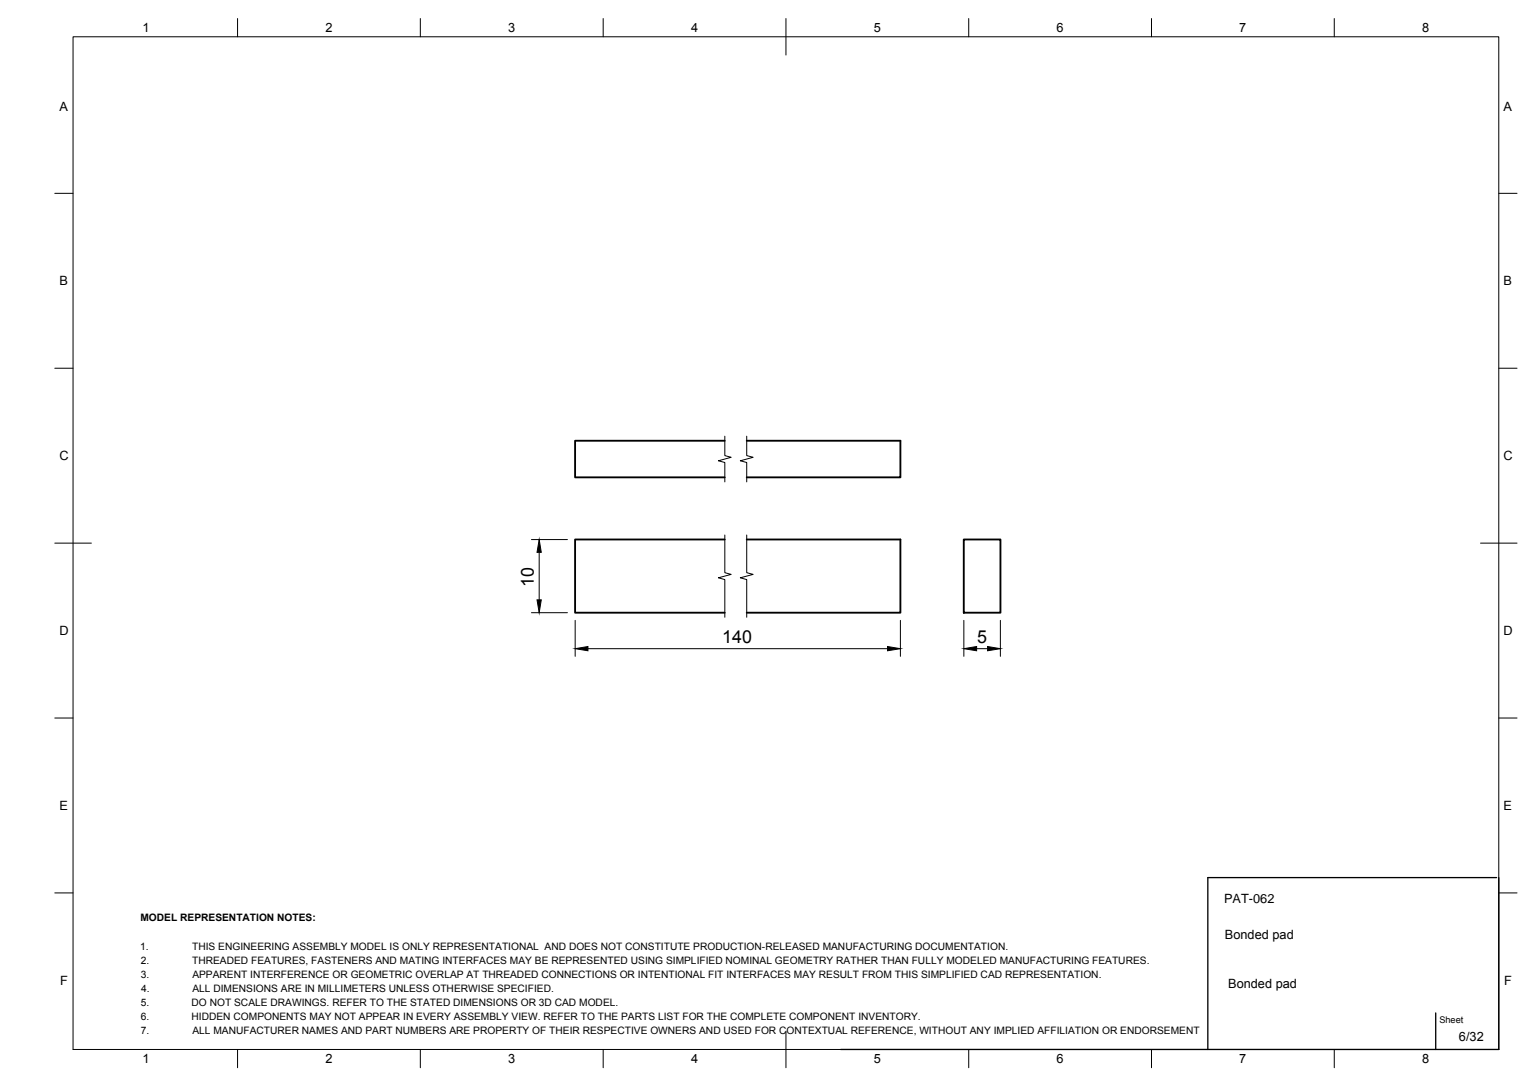
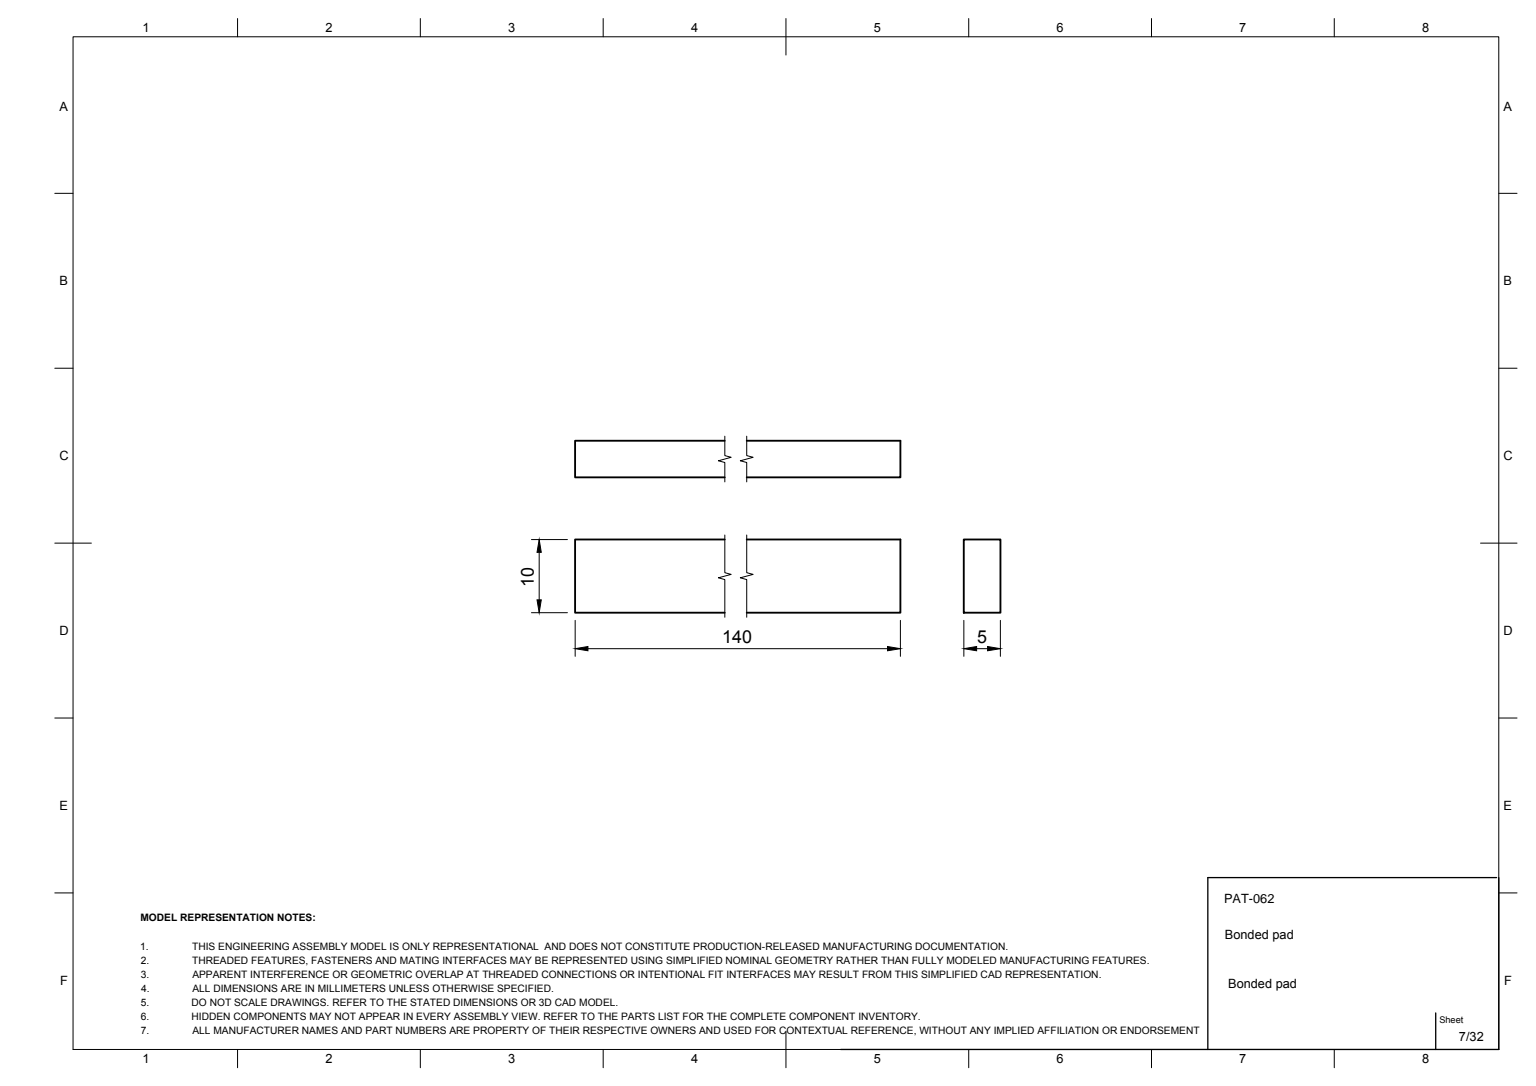
ISO-10303-21;
HEADER;
/* Generated by software containing ST-Developer
 * from STEP Tools, Inc. (www.steptools.com) 
 */

FILE_DESCRIPTION(
/* description */ ('Jaw-coupled motor to shaft test stand'),
/* implementation_level */ '2;1');

FILE_NAME(
/* name */ 'Bonded pad.step',
/* time_stamp */ '2026-10-27T10:46:06-07:00',
/* author */ (''),
/* organization */ (''),
/* preprocessor_version */ 'ST-DEVELOPER v20.2',
/* originating_system */ 'Autodesk Translation Framework v15.17.0.0',
/* authorisation */ '');

FILE_SCHEMA (('AUTOMOTIVE_DESIGN { 1 0 10303 214 3 1 1 }'));
ENDSEC;

DATA;
#10=MECHANICAL_DESIGN_GEOMETRIC_PRESENTATION_REPRESENTATION('',(#341),#19361);
#277=SHAPE_REPRESENTATION_RELATIONSHIP('SRR','None',#19491,#309);
#309=ADVANCED_BREP_SHAPE_REPRESENTATION('',(#374),#19327);
#341=STYLED_ITEM('',(#19760),#374);
#374=MANIFOLD_SOLID_BREP('Body1',#10985);
#522=PLANE('',#11401);
#523=PLANE('',#11402);
#524=PLANE('',#11403);
#525=PLANE('',#11404);
#526=PLANE('',#11405);
#527=PLANE('',#11406);
#1034=FACE_OUTER_BOUND('',#1666,.T.);
#1035=FACE_OUTER_BOUND('',#1667,.T.);
#1036=FACE_OUTER_BOUND('',#1668,.T.);
#1037=FACE_OUTER_BOUND('',#1669,.T.);
#1038=FACE_OUTER_BOUND('',#1670,.T.);
#1039=FACE_OUTER_BOUND('',#1671,.T.);
#1666=EDGE_LOOP('',(#7406,#7407,#7408,#7409));
#1667=EDGE_LOOP('',(#7410,#7411,#7412,#7413));
#1668=EDGE_LOOP('',(#7414,#7415,#7416,#7417));
#1669=EDGE_LOOP('',(#7418,#7419,#7420,#7421));
#1670=EDGE_LOOP('',(#7422,#7423,#7424,#7425));
#1671=EDGE_LOOP('',(#7426,#7427,#7428,#7429));
#2393=LINE('',#15496,#3546);
#2394=LINE('',#15498,#3547);
#2395=LINE('',#15500,#3548);
#2396=LINE('',#15501,#3549);
#2397=LINE('',#15504,#3550);
#2398=LINE('',#15506,#3551);
#2399=LINE('',#15507,#3552);
#2400=LINE('',#15510,#3553);
#2401=LINE('',#15512,#3554);
#2402=LINE('',#15513,#3555);
#2403=LINE('',#15515,#3556);
#2404=LINE('',#15516,#3557);
#3546=VECTOR('',#12416,1.);
#3547=VECTOR('',#12417,1.);
#3548=VECTOR('',#12418,1.);
#3549=VECTOR('',#12419,1.);
#3550=VECTOR('',#12422,1.);
#3551=VECTOR('',#12423,1.);
#3552=VECTOR('',#12424,1.);
#3553=VECTOR('',#12427,1.);
#3554=VECTOR('',#12428,1.);
#3555=VECTOR('',#12429,1.);
#3556=VECTOR('',#12432,1.);
#3557=VECTOR('',#12433,1.);
#4963=VERTEX_POINT('',#15494);
#4964=VERTEX_POINT('',#15495);
#4965=VERTEX_POINT('',#15497);
#4966=VERTEX_POINT('',#15499);
#4967=VERTEX_POINT('',#15503);
#4968=VERTEX_POINT('',#15505);
#4969=VERTEX_POINT('',#15509);
#4970=VERTEX_POINT('',#15511);
#5914=EDGE_CURVE('',#4963,#4964,#2393,.T.);
#5915=EDGE_CURVE('',#4964,#4965,#2394,.T.);
#5916=EDGE_CURVE('',#4966,#4965,#2395,.T.);
#5917=EDGE_CURVE('',#4963,#4966,#2396,.T.);
#5918=EDGE_CURVE('',#4967,#4963,#2397,.T.);
#5919=EDGE_CURVE('',#4968,#4966,#2398,.T.);
#5920=EDGE_CURVE('',#4967,#4968,#2399,.T.);
#5921=EDGE_CURVE('',#4969,#4967,#2400,.T.);
#5922=EDGE_CURVE('',#4970,#4968,#2401,.T.);
#5923=EDGE_CURVE('',#4969,#4970,#2402,.T.);
#5924=EDGE_CURVE('',#4964,#4969,#2403,.T.);
#5925=EDGE_CURVE('',#4965,#4970,#2404,.T.);
#7406=ORIENTED_EDGE('',*,*,#5914,.T.);
#7407=ORIENTED_EDGE('',*,*,#5915,.T.);
#7408=ORIENTED_EDGE('',*,*,#5916,.F.);
#7409=ORIENTED_EDGE('',*,*,#5917,.F.);
#7410=ORIENTED_EDGE('',*,*,#5918,.T.);
#7411=ORIENTED_EDGE('',*,*,#5917,.T.);
#7412=ORIENTED_EDGE('',*,*,#5919,.F.);
#7413=ORIENTED_EDGE('',*,*,#5920,.F.);
#7414=ORIENTED_EDGE('',*,*,#5921,.T.);
#7415=ORIENTED_EDGE('',*,*,#5920,.T.);
#7416=ORIENTED_EDGE('',*,*,#5922,.F.);
#7417=ORIENTED_EDGE('',*,*,#5923,.F.);
#7418=ORIENTED_EDGE('',*,*,#5924,.T.);
#7419=ORIENTED_EDGE('',*,*,#5923,.T.);
#7420=ORIENTED_EDGE('',*,*,#5925,.F.);
#7421=ORIENTED_EDGE('',*,*,#5915,.F.);
#7422=ORIENTED_EDGE('',*,*,#5925,.T.);
#7423=ORIENTED_EDGE('',*,*,#5922,.T.);
#7424=ORIENTED_EDGE('',*,*,#5919,.T.);
#7425=ORIENTED_EDGE('',*,*,#5916,.T.);
#7426=ORIENTED_EDGE('',*,*,#5924,.F.);
#7427=ORIENTED_EDGE('',*,*,#5914,.F.);
#7428=ORIENTED_EDGE('',*,*,#5918,.F.);
#7429=ORIENTED_EDGE('',*,*,#5921,.F.);
#10376=ADVANCED_FACE('',(#1034),#522,.T.);
#10377=ADVANCED_FACE('',(#1035),#523,.T.);
#10378=ADVANCED_FACE('',(#1036),#524,.T.);
#10379=ADVANCED_FACE('',(#1037),#525,.T.);
#10380=ADVANCED_FACE('',(#1038),#526,.T.);
#10381=ADVANCED_FACE('',(#1039),#527,.F.);
#10985=CLOSED_SHELL('',(#10376,#10377,#10378,#10379,#10380,#10381));
#11400=AXIS2_PLACEMENT_3D('',#15492,#12412,#12413);
#11401=AXIS2_PLACEMENT_3D('',#15493,#12414,#12415);
#11402=AXIS2_PLACEMENT_3D('',#15502,#12420,#12421);
#11403=AXIS2_PLACEMENT_3D('',#15508,#12425,#12426);
#11404=AXIS2_PLACEMENT_3D('',#15514,#12430,#12431);
#11405=AXIS2_PLACEMENT_3D('',#15517,#12434,#12435);
#11406=AXIS2_PLACEMENT_3D('',#15518,#12436,#12437);
#12412=DIRECTION('axis',(0.,0.,1.));
#12413=DIRECTION('refdir',(1.,0.,0.));
#12414=DIRECTION('center_axis',(0.,1.,0.));
#12415=DIRECTION('ref_axis',(-1.,0.,0.));
#12416=DIRECTION('',(-1.,0.,0.));
#12417=DIRECTION('',(0.,0.,1.));
#12418=DIRECTION('',(-1.,0.,0.));
#12419=DIRECTION('',(0.,0.,1.));
#12420=DIRECTION('center_axis',(1.,0.,0.));
#12421=DIRECTION('ref_axis',(0.,1.,0.));
#12422=DIRECTION('',(0.,1.,0.));
#12423=DIRECTION('',(0.,1.,0.));
#12424=DIRECTION('',(0.,0.,1.));
#12425=DIRECTION('center_axis',(0.,-1.,0.));
#12426=DIRECTION('ref_axis',(1.,0.,0.));
#12427=DIRECTION('',(1.,0.,0.));
#12428=DIRECTION('',(1.,0.,0.));
#12429=DIRECTION('',(0.,0.,1.));
#12430=DIRECTION('center_axis',(-1.,0.,0.));
#12431=DIRECTION('ref_axis',(0.,-1.,0.));
#12432=DIRECTION('',(0.,-1.,0.));
#12433=DIRECTION('',(0.,-1.,0.));
#12434=DIRECTION('center_axis',(0.,0.,1.));
#12435=DIRECTION('ref_axis',(1.,0.,0.));
#12436=DIRECTION('center_axis',(0.,0.,1.));
#12437=DIRECTION('ref_axis',(1.,0.,0.));
#15492=CARTESIAN_POINT('',(0.,0.,0.));
#15493=CARTESIAN_POINT('Origin',(7.,-11.5,-0.5));
#15494=CARTESIAN_POINT('',(7.,-11.5,-0.5));
#15495=CARTESIAN_POINT('',(-7.,-11.5,-0.5));
#15496=CARTESIAN_POINT('',(7.,-11.5,-0.5));
#15497=CARTESIAN_POINT('',(-7.,-11.5,0.));
#15498=CARTESIAN_POINT('',(-7.,-11.5,-0.5));
#15499=CARTESIAN_POINT('',(7.,-11.5,0.));
#15500=CARTESIAN_POINT('',(7.,-11.5,0.));
#15501=CARTESIAN_POINT('',(7.,-11.5,-0.5));
#15502=CARTESIAN_POINT('Origin',(7.,-12.5,-0.5));
#15503=CARTESIAN_POINT('',(7.,-12.5,-0.5));
#15504=CARTESIAN_POINT('',(7.,-12.5,-0.5));
#15505=CARTESIAN_POINT('',(7.,-12.5,0.));
#15506=CARTESIAN_POINT('',(7.,-12.5,0.));
#15507=CARTESIAN_POINT('',(7.,-12.5,-0.5));
#15508=CARTESIAN_POINT('Origin',(-7.,-12.5,-0.5));
#15509=CARTESIAN_POINT('',(-7.,-12.5,-0.5));
#15510=CARTESIAN_POINT('',(-7.,-12.5,-0.5));
#15511=CARTESIAN_POINT('',(-7.,-12.5,0.));
#15512=CARTESIAN_POINT('',(-7.,-12.5,0.));
#15513=CARTESIAN_POINT('',(-7.,-12.5,-0.5));
#15514=CARTESIAN_POINT('Origin',(-7.,-11.5,-0.5));
#15515=CARTESIAN_POINT('',(-7.,-11.5,-0.5));
#15516=CARTESIAN_POINT('',(-7.,-11.5,0.));
#15517=CARTESIAN_POINT('Origin',(0.,-12.,0.));
#15518=CARTESIAN_POINT('Origin',(0.,-12.,-0.5));
#19289=UNCERTAINTY_MEASURE_WITH_UNIT(LENGTH_MEASURE(0.001),#19362,
'DISTANCE_ACCURACY_VALUE',
'Maximum model space distance between geometric entities at asserted c
onnectivities');
#19323=UNCERTAINTY_MEASURE_WITH_UNIT(LENGTH_MEASURE(0.001),#19362,
'DISTANCE_ACCURACY_VALUE',
'Maximum model space distance between geometric entities at asserted c
onnectivities');
#19327=(
GEOMETRIC_REPRESENTATION_CONTEXT(3)
GLOBAL_UNCERTAINTY_ASSIGNED_CONTEXT((#19289))
GLOBAL_UNIT_ASSIGNED_CONTEXT((#19362,#19364,#19365))
REPRESENTATION_CONTEXT('','3D')
);
#19361=(
GEOMETRIC_REPRESENTATION_CONTEXT(3)
GLOBAL_UNCERTAINTY_ASSIGNED_CONTEXT((#19323))
GLOBAL_UNIT_ASSIGNED_CONTEXT((#19362,#19364,#19365))
REPRESENTATION_CONTEXT('','3D')
);
#19362=(
LENGTH_UNIT()
NAMED_UNIT(*)
SI_UNIT(.CENTI.,.METRE.)
);
#19364=(
NAMED_UNIT(*)
PLANE_ANGLE_UNIT()
SI_UNIT($,.RADIAN.)
);
#19365=(
NAMED_UNIT(*)
SI_UNIT($,.STERADIAN.)
SOLID_ANGLE_UNIT()
);
#19369=SHAPE_DEFINITION_REPRESENTATION(#19406,#19491);
#19406=PRODUCT_DEFINITION_SHAPE('',$,#19529);
#19491=SHAPE_REPRESENTATION('',(#11400),#19327);
#19525=PRODUCT_DEFINITION_CONTEXT('part definition',#19638,'design');
#19529=PRODUCT_DEFINITION('Bonded pad','Bonded pad',#19566,#19525);
#19566=PRODUCT_DEFINITION_FORMATION('',$,#19643);
#19638=APPLICATION_CONTEXT(
'Core Data for Automotive Mechanical Design Process');
#19639=PRODUCT_CONTEXT('part definition',#19638,'mechanical');
#19643=PRODUCT('Bonded pad','Bonded pad','Bonded pad',(#19639));
#19754=COLOUR_RGB('Off White',0.89,0.88,0.83);
#19755=FILL_AREA_STYLE_COLOUR('',#19754);
#19756=FILL_AREA_STYLE('',(#19755));
#19757=SURFACE_STYLE_FILL_AREA(#19756);
#19758=SURFACE_SIDE_STYLE('',(#19757));
#19759=SURFACE_STYLE_USAGE(.BOTH.,#19758);
#19760=PRESENTATION_STYLE_ASSIGNMENT((#19759));
ENDSEC;
END-ISO-10303-21;
